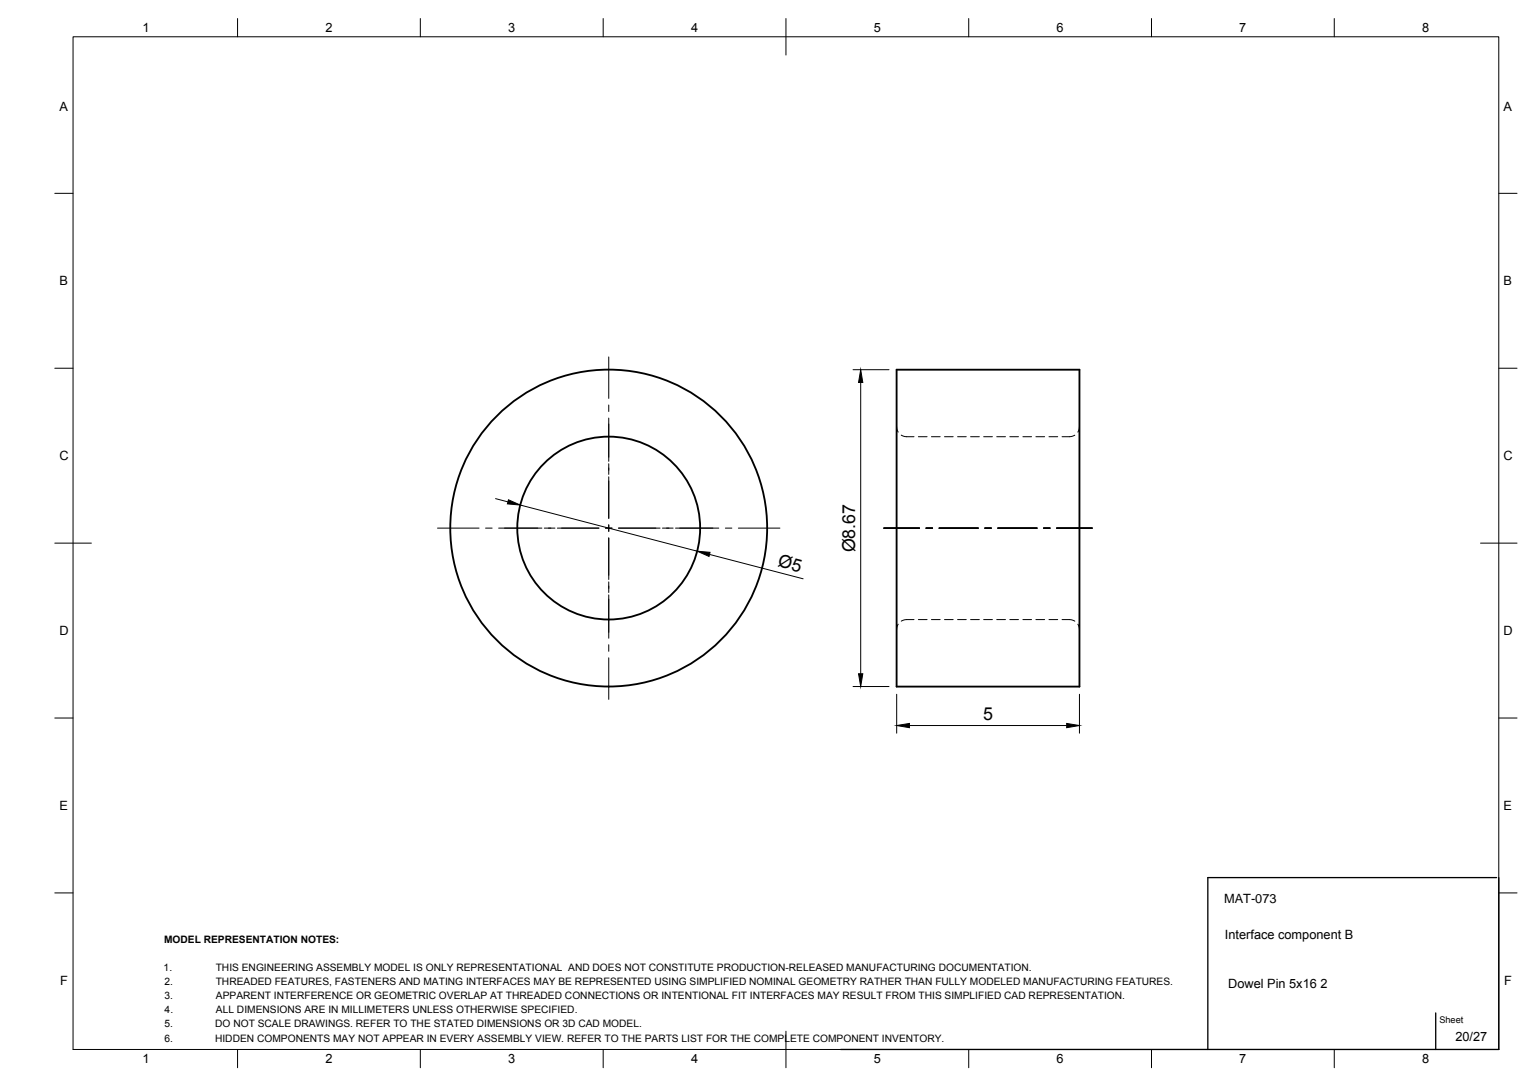
ISO-10303-21;
HEADER;
/* Generated by software containing ST-Developer
 * from STEP Tools, Inc. (www.steptools.com) 
 */

FILE_DESCRIPTION(
/* description */ ('CAx-IF Rec.Pracs.---Representation and Presentation of Product Manufa
cturing Information (PMI)---4.0---2014-10-13'),
/* implementation_level */ '2;1');

FILE_NAME(
/* name */ 'Interface component B.step',
/* time_stamp */ '2026-10-24T18:52:33-07:00',
/* author */ (''),
/* organization */ (''),
/* preprocessor_version */ 'ST-DEVELOPER v20.2',
/* originating_system */ 'Autodesk Translation Framework v15.17.0.0',
/* authorisation */ '');

FILE_SCHEMA (('AP242_MANAGED_MODEL_BASED_3D_ENGINEERING_MIM_LF { 1 0 10303 442 2 1 4 }'));
ENDSEC;

DATA;
#10=MECHANICAL_DESIGN_GEOMETRIC_PRESENTATION_REPRESENTATION('',(#435),#34876);
#369=SHAPE_REPRESENTATION_RELATIONSHIP('SRR','None',#35006,#402);
#402=ADVANCED_BREP_SHAPE_REPRESENTATION('',(#468),#34864);
#435=STYLED_ITEM('',(#35163),#468);
#468=MANIFOLD_SOLID_BREP('Dowel Pin 5x16 2',#19575);
#560=FACE_BOUND('',#6674,.T.);
#561=FACE_BOUND('',#6677,.T.);
#927=PLANE('',#21659);
#928=PLANE('',#21664);
#2174=LINE('',#32942,#3773);
#2175=LINE('',#32955,#3774);
#3773=VECTOR('',#26763,0.0025);
#3774=VECTOR('',#26782,0.00433333333333334);
#4679=CYLINDRICAL_SURFACE('',#21656,0.0025);
#4680=CYLINDRICAL_SURFACE('',#21666,0.00433333333333334);
#5546=FACE_OUTER_BOUND('',#6671,.T.);
#5547=FACE_OUTER_BOUND('',#6672,.T.);
#5548=FACE_OUTER_BOUND('',#6673,.T.);
#5549=FACE_OUTER_BOUND('',#6675,.T.);
#5550=FACE_OUTER_BOUND('',#6676,.T.);
#5551=FACE_OUTER_BOUND('',#6678,.T.);
#6671=EDGE_LOOP('',(#16880,#16881,#16882,#16883,#16884));
#6672=EDGE_LOOP('',(#16885,#16886,#16887,#16888,#16889,#16890));
#6673=EDGE_LOOP('',(#16891));
#6674=EDGE_LOOP('',(#16892));
#6675=EDGE_LOOP('',(#16893,#16894,#16895,#16896,#16897));
#6676=EDGE_LOOP('',(#16898));
#6677=EDGE_LOOP('',(#16899));
#6678=EDGE_LOOP('',(#16900,#16901,#16902,#16903));
#7805=CIRCLE('',#21652,0.00250000000001);
#7806=CIRCLE('',#21653,0.000275);
#7807=CIRCLE('',#21654,0.00277500000001);
#7808=CIRCLE('',#21655,0.00250000000001);
#7809=CIRCLE('',#21657,0.00250000000001);
#7810=CIRCLE('',#21658,0.00250000000001);
#7811=CIRCLE('',#21660,0.00433333333334334);
#7812=CIRCLE('',#21662,0.00277500000001);
#7813=CIRCLE('',#21663,0.000275);
#7814=CIRCLE('',#21665,0.00433333333334334);
#9423=VERTEX_POINT('',#32931);
#9424=VERTEX_POINT('',#32932);
#9425=VERTEX_POINT('',#32934);
#9426=VERTEX_POINT('',#32939);
#9427=VERTEX_POINT('',#32940);
#9428=VERTEX_POINT('',#32945);
#9429=VERTEX_POINT('',#32948);
#9430=VERTEX_POINT('',#32952);
#11998=EDGE_CURVE('',#9423,#9424,#7805,.T.);
#11999=EDGE_CURVE('',#9424,#9425,#7806,.T.);
#12000=EDGE_CURVE('',#9425,#9425,#7807,.T.);
#12001=EDGE_CURVE('',#9424,#9423,#7808,.T.);
#12002=EDGE_CURVE('',#9426,#9427,#7809,.T.);
#12003=EDGE_CURVE('',#9426,#9423,#2174,.T.);
#12004=EDGE_CURVE('',#9427,#9426,#7810,.T.);
#12005=EDGE_CURVE('',#9428,#9428,#7811,.T.);
#12006=EDGE_CURVE('',#9429,#9429,#7812,.T.);
#12007=EDGE_CURVE('',#9429,#9427,#7813,.T.);
#12008=EDGE_CURVE('',#9430,#9430,#7814,.T.);
#12009=EDGE_CURVE('',#9428,#9430,#2175,.T.);
#16880=ORIENTED_EDGE('',*,*,#11998,.T.);
#16881=ORIENTED_EDGE('',*,*,#11999,.T.);
#16882=ORIENTED_EDGE('',*,*,#12000,.T.);
#16883=ORIENTED_EDGE('',*,*,#11999,.F.);
#16884=ORIENTED_EDGE('',*,*,#12001,.T.);
#16885=ORIENTED_EDGE('',*,*,#12002,.F.);
#16886=ORIENTED_EDGE('',*,*,#12003,.T.);
#16887=ORIENTED_EDGE('',*,*,#12001,.F.);
#16888=ORIENTED_EDGE('',*,*,#11998,.F.);
#16889=ORIENTED_EDGE('',*,*,#12003,.F.);
#16890=ORIENTED_EDGE('',*,*,#12004,.F.);
#16891=ORIENTED_EDGE('',*,*,#12005,.T.);
#16892=ORIENTED_EDGE('',*,*,#12000,.F.);
#16893=ORIENTED_EDGE('',*,*,#12006,.T.);
#16894=ORIENTED_EDGE('',*,*,#12007,.T.);
#16895=ORIENTED_EDGE('',*,*,#12004,.T.);
#16896=ORIENTED_EDGE('',*,*,#12002,.T.);
#16897=ORIENTED_EDGE('',*,*,#12007,.F.);
#16898=ORIENTED_EDGE('',*,*,#12008,.F.);
#16899=ORIENTED_EDGE('',*,*,#12006,.F.);
#16900=ORIENTED_EDGE('',*,*,#12005,.F.);
#16901=ORIENTED_EDGE('',*,*,#12009,.T.);
#16902=ORIENTED_EDGE('',*,*,#12008,.T.);
#16903=ORIENTED_EDGE('',*,*,#12009,.F.);
#18500=TOROIDAL_SURFACE('',#21651,0.002775,0.000275);
#18501=TOROIDAL_SURFACE('',#21661,0.002775,0.000275);
#19262=ADVANCED_FACE('',(#5546),#18500,.T.);
#19263=ADVANCED_FACE('',(#5547),#4679,.F.);
#19264=ADVANCED_FACE('',(#5548,#560),#927,.T.);
#19265=ADVANCED_FACE('',(#5549),#18501,.T.);
#19266=ADVANCED_FACE('',(#5550,#561),#928,.T.);
#19267=ADVANCED_FACE('',(#5551),#4680,.T.);
#19575=CLOSED_SHELL('',(#19262,#19263,#19264,#19265,#19266,#19267));
#21650=AXIS2_PLACEMENT_3D('',#32929,#26747,#26748);
#21651=AXIS2_PLACEMENT_3D('',#32930,#26749,#26750);
#21652=AXIS2_PLACEMENT_3D('',#32933,#26751,#26752);
#21653=AXIS2_PLACEMENT_3D('',#32935,#26753,#26754);
#21654=AXIS2_PLACEMENT_3D('',#32936,#26755,#26756);
#21655=AXIS2_PLACEMENT_3D('',#32937,#26757,#26758);
#21656=AXIS2_PLACEMENT_3D('',#32938,#26759,#26760);
#21657=AXIS2_PLACEMENT_3D('',#32941,#26761,#26762);
#21658=AXIS2_PLACEMENT_3D('',#32943,#26764,#26765);
#21659=AXIS2_PLACEMENT_3D('',#32944,#26766,#26767);
#21660=AXIS2_PLACEMENT_3D('',#32946,#26768,#26769);
#21661=AXIS2_PLACEMENT_3D('',#32947,#26770,#26771);
#21662=AXIS2_PLACEMENT_3D('',#32949,#26772,#26773);
#21663=AXIS2_PLACEMENT_3D('',#32950,#26774,#26775);
#21664=AXIS2_PLACEMENT_3D('',#32951,#26776,#26777);
#21665=AXIS2_PLACEMENT_3D('',#32953,#26778,#26779);
#21666=AXIS2_PLACEMENT_3D('',#32954,#26780,#26781);
#26747=DIRECTION('axis',(0.,0.,1.));
#26748=DIRECTION('refdir',(1.,0.,0.));
#26749=DIRECTION('center_axis',(6.12323404134149E-17,-1.,3.14444500472474E-32));
#26750=DIRECTION('ref_axis',(1.55749764652046E-5,0.,-0.99999999987871));
#26751=DIRECTION('center_axis',(-6.12323404134149E-17,1.,-3.14444500472474E-32));
#26752=DIRECTION('ref_axis',(-0.99999999987871,-6.1232340405988E-17,-1.55749724650822E-5));
#26753=DIRECTION('center_axis',(-0.99999999987871,-6.1232340405988E-17,
-1.55749764653271E-5));
#26754=DIRECTION('ref_axis',(-1.55749764653271E-5,0.,0.99999999987871));
#26755=DIRECTION('center_axis',(6.12323404134149E-17,-1.,3.14444500472474E-32));
#26756=DIRECTION('ref_axis',(-0.99999999987871,-6.1232340405988E-17,-1.55749728614786E-5));
#26757=DIRECTION('center_axis',(-6.12323404134149E-17,1.,-3.14444500472474E-32));
#26758=DIRECTION('ref_axis',(-0.99999999987871,-6.1232340405988E-17,-1.55749724650822E-5));
#26759=DIRECTION('center_axis',(6.12323404134149E-17,-1.,3.14444500472474E-32));
#26760=DIRECTION('ref_axis',(0.99999999987871,6.1232340405988E-17,1.55749764652046E-5));
#26761=DIRECTION('center_axis',(6.12323404134149E-17,-1.,3.14444500472474E-32));
#26762=DIRECTION('ref_axis',(-0.99999999987871,-6.1232340405988E-17,-1.55749724650822E-5));
#26763=DIRECTION('',(6.12323404134149E-17,-1.,3.14444500472474E-32));
#26764=DIRECTION('center_axis',(6.12323404134149E-17,-1.,3.14444500472474E-32));
#26765=DIRECTION('ref_axis',(-0.99999999987871,-6.1232340405988E-17,-1.55749724650822E-5));
#26766=DIRECTION('center_axis',(6.12323404134149E-17,-1.,3.14444500472474E-32));
#26767=DIRECTION('ref_axis',(0.99999999987871,6.12323404059881E-17,1.55749764652046E-5));
#26768=DIRECTION('center_axis',(6.12323404134149E-17,-1.,3.14444500472474E-32));
#26769=DIRECTION('ref_axis',(0.99999999987871,6.1232340405988E-17,1.55749764652046E-5));
#26770=DIRECTION('center_axis',(6.12323404134149E-17,-1.,3.14444500472474E-32));
#26771=DIRECTION('ref_axis',(1.55749764652046E-5,0.,-0.99999999987871));
#26772=DIRECTION('center_axis',(-6.12323404134149E-17,1.,-3.14444500472474E-32));
#26773=DIRECTION('ref_axis',(-0.99999999987871,-6.1232340405988E-17,-1.55749728614786E-5));
#26774=DIRECTION('center_axis',(-0.99999999987871,-6.1232340405988E-17,
-1.55749764653271E-5));
#26775=DIRECTION('ref_axis',(-1.55749764653271E-5,0.,0.99999999987871));
#26776=DIRECTION('center_axis',(-6.12323404134149E-17,1.,-3.14444500472474E-32));
#26777=DIRECTION('ref_axis',(-1.55749764652046E-5,-9.53692260816889E-22,
0.99999999987871));
#26778=DIRECTION('center_axis',(6.12323404134149E-17,-1.,3.14444500472474E-32));
#26779=DIRECTION('ref_axis',(0.99999999987871,6.1232340405988E-17,1.55749764652046E-5));
#26780=DIRECTION('center_axis',(6.12323404134149E-17,-1.,3.14444500472474E-32));
#26781=DIRECTION('ref_axis',(0.99999999987871,6.1232340405988E-17,1.55749764652046E-5));
#26782=DIRECTION('',(-6.12323404134149E-17,1.,-3.14444500472474E-32));
#32929=CARTESIAN_POINT('',(0.,0.,0.));
#32930=CARTESIAN_POINT('Origin',(-4.34919666873154E-17,-0.030975,7.19534755436855E-33));
#32931=CARTESIAN_POINT('',(-0.00249999999970682,-0.03097500000001,-3.89374311628611E-8));
#32932=CARTESIAN_POINT('',(-3.89374412069654E-8,-0.03097500000001,0.00249999999970677));
#32933=CARTESIAN_POINT('Origin',(-4.34919666873148E-17,-0.03097500000001,
7.19534755436887E-33));
#32934=CARTESIAN_POINT('',(-4.32205597349135E-8,-0.03125000000001,0.00277499999967342));
#32935=CARTESIAN_POINT('Origin',(-4.32205597347746E-8,-0.030975,0.00277499999966342));
#32936=CARTESIAN_POINT('Origin',(-4.34751277937011E-17,-0.03125000000001,
7.20399477813186E-33));
#32937=CARTESIAN_POINT('Origin',(-4.34919666873148E-17,-0.03097500000001,
7.19534755436887E-33));
#32938=CARTESIAN_POINT('Origin',(-4.36282086447352E-17,-0.02875,7.12538365301343E-33));
#32939=CARTESIAN_POINT('',(-0.00249999999970682,-0.02652500000001,-3.89374311628611E-8));
#32940=CARTESIAN_POINT('',(-3.89374412072379E-8,-0.02652500000001,0.00249999999970677));
#32941=CARTESIAN_POINT('Origin',(-4.37644506021545E-17,-0.02652500000001,
7.05541975165862E-33));
#32942=CARTESIAN_POINT('',(-0.00249999999969682,-0.02875,-3.89374411633177E-8));
#32943=CARTESIAN_POINT('Origin',(-4.37644506021545E-17,-0.02652500000001,
7.05541975165862E-33));
#32944=CARTESIAN_POINT('Origin',(0.00341666666625222,-0.03125,5.32145029227824E-8));
#32945=CARTESIAN_POINT('',(-0.0043333333328078,-0.03125000000001,-6.74915646830841E-8));
#32946=CARTESIAN_POINT('Origin',(-4.34751277937011E-17,-0.03125000000001,
7.20399477813186E-33));
#32947=CARTESIAN_POINT('Origin',(-4.37644506021551E-17,-0.026525,7.0554197516583E-33));
#32948=CARTESIAN_POINT('',(-4.32205597352196E-8,-0.02625000000001,0.00277499999967342));
#32949=CARTESIAN_POINT('Origin',(-4.37812894957682E-17,-0.02625000000001,
7.04677252789562E-33));
#32950=CARTESIAN_POINT('Origin',(-4.32205597350471E-8,-0.026525,0.00277499999966342));
#32951=CARTESIAN_POINT('Origin',(0.00341666666625222,-0.02625,5.32145029227824E-8));
#32952=CARTESIAN_POINT('',(-0.0043333333328078,-0.02625000000001,-6.74915646830841E-8));
#32953=CARTESIAN_POINT('Origin',(-4.37812894957682E-17,-0.02625000000001,
7.04677252789562E-33));
#32954=CARTESIAN_POINT('Origin',(-4.36282086447352E-17,-0.02875,7.12538365301343E-33));
#32955=CARTESIAN_POINT('',(-0.0043333333328078,-0.02875,-6.74915646830841E-8));
#34829=UNCERTAINTY_MEASURE_WITH_UNIT(LENGTH_MEASURE(1.E-5),#34877,
'DISTANCE_ACCURACY_VALUE',
'Maximum model space distance between geometric entities at asserted c
onnectivities');
#34841=UNCERTAINTY_MEASURE_WITH_UNIT(LENGTH_MEASURE(1.E-5),#34877,
'DISTANCE_ACCURACY_VALUE',
'Maximum model space distance between geometric entities at asserted c
onnectivities');
#34864=(
GEOMETRIC_REPRESENTATION_CONTEXT(3)
GLOBAL_UNCERTAINTY_ASSIGNED_CONTEXT((#34829))
GLOBAL_UNIT_ASSIGNED_CONTEXT((#34877,#34878,#34879))
REPRESENTATION_CONTEXT('','3D')
);
#34876=(
GEOMETRIC_REPRESENTATION_CONTEXT(3)
GLOBAL_UNCERTAINTY_ASSIGNED_CONTEXT((#34841))
GLOBAL_UNIT_ASSIGNED_CONTEXT((#34877,#34878,#34879))
REPRESENTATION_CONTEXT('','3D')
);
#34877=(
LENGTH_UNIT()
NAMED_UNIT(*)
SI_UNIT($,.METRE.)
);
#34878=(
NAMED_UNIT(*)
PLANE_ANGLE_UNIT()
SI_UNIT($,.RADIAN.)
);
#34879=(
NAMED_UNIT(*)
SI_UNIT($,.STERADIAN.)
SOLID_ANGLE_UNIT()
);
#34902=SHAPE_DEFINITION_REPRESENTATION(#34936,#35006);
#34936=PRODUCT_DEFINITION_SHAPE('',$,#35041);
#35006=SHAPE_REPRESENTATION('',(#21650),#34864);
#35018=PRODUCT_DEFINITION_CONTEXT('part definition',#35122,'design');
#35041=PRODUCT_DEFINITION('Interface component B',
'Interface component B',#35075,#35018);
#35075=PRODUCT_DEFINITION_FORMATION('',$,#35146);
#35122=APPLICATION_CONTEXT('Managed model based 3d engineering');
#35123=PRODUCT_CONTEXT('part definition',#35122,'mechanical');
#35146=PRODUCT('Interface component B','Interface component B',
'LEGAL AND USAGE DISCLAIMER: this Data/Model is provided \X2\201C\X0\A
S IS\X2\201D\X0\ for informational and representational only. It is a 
geometric approximation and is NOT engineered, certified, or guarantee
d for dimensional accuracy, exact tolerances, or production-level prec
ision. Vendor disclaims all implied warranties including fitness for a
 particular purpose. DO NOT USE FOR DIRECT PHYSICAL MANUFACTURING, AUT
OMATED PRODUCTION, OR SAFETY-CRITICAL SYSTEMS without independent engi
neering verification and resolution of any design discrepancies.',(#35123));
#35163=PRESENTATION_STYLE_ASSIGNMENT((#35172));
#35172=SURFACE_STYLE_USAGE(.BOTH.,#35181);
#35181=SURFACE_SIDE_STYLE('',(#35190));
#35190=SURFACE_STYLE_FILL_AREA(#35199);
#35199=FILL_AREA_STYLE('Plastic - Matte (Black)',(#35208));
#35208=FILL_AREA_STYLE_COLOUR('Plastic - Matte (Black)',#35217);
#35217=COLOUR_RGB('Plastic - Matte (Black)',0.0980392156862745,0.0980392156862745,
0.0980392156862745);
ENDSEC;
END-ISO-10303-21;
